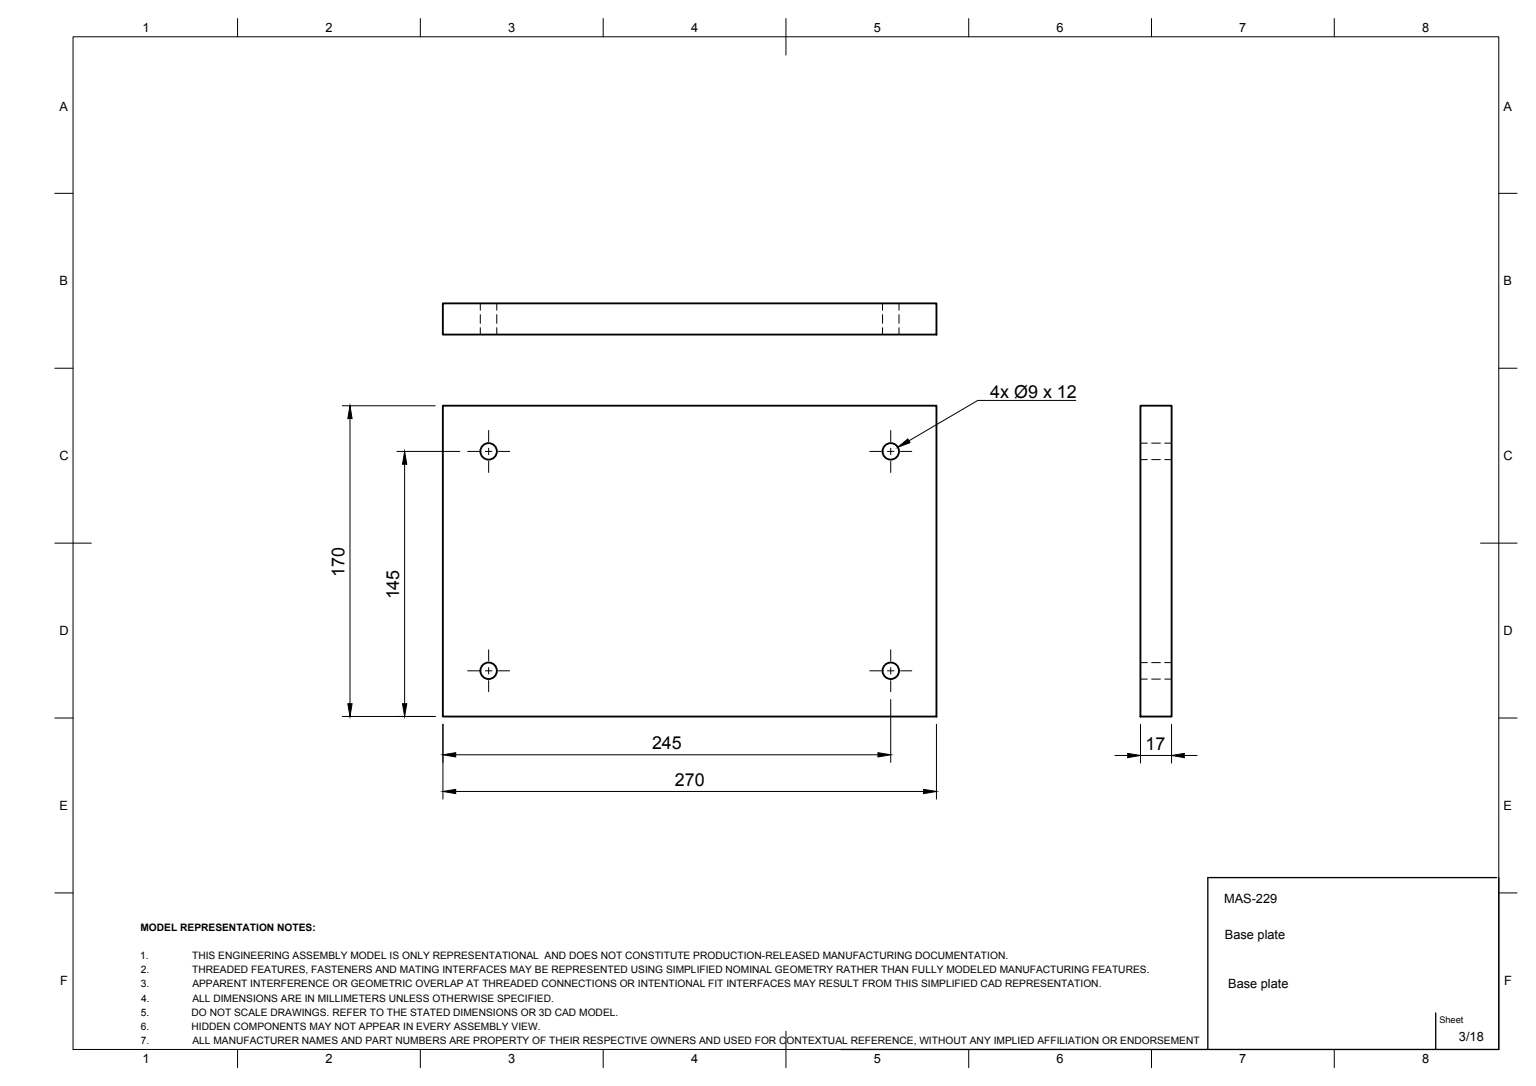
ISO-10303-21;
HEADER;
/* Generated by software containing ST-Developer
 * from STEP Tools, Inc. (www.steptools.com) 
 */

FILE_DESCRIPTION(
/* description */ ('Independently dimensioned six-bar single-leg walking-linkage demonstr
ator. Whole-mm20 crank,60 upper rocker,80/120 ternary coupler,120 lowe
r rocker,140 knee pitch and260 toe reach; ground pivots0/0,60/0,40/60.
 Seven native revolutes close both loops. Four reused native library f
amilies, fully retained shared pins and layered real spacer stacks, bo
nded rubber toe. Benchtop reference mechanism; no complete vehicle, lo
ad, gait stability, adhesive, weld, fit or life rating.'),
/* implementation_level */ '2;1');

FILE_NAME(
/* name */ 'Base plate.step',
/* time_stamp */ '2026-11-09T20:33:14-08:00',
/* author */ (''),
/* organization */ (''),
/* preprocessor_version */ 'ST-DEVELOPER v20.2',
/* originating_system */ 'Autodesk Translation Framework v15.17.0.0',
/* authorisation */ '');

FILE_SCHEMA (('AUTOMOTIVE_DESIGN { 1 0 10303 214 3 1 1 }'));
ENDSEC;

DATA;
#10=MECHANICAL_DESIGN_GEOMETRIC_PRESENTATION_REPRESENTATION('',(#255),#4048);
#219=SHAPE_REPRESENTATION_RELATIONSHIP('SRR','None',#4143,#237);
#237=ADVANCED_BREP_SHAPE_REPRESENTATION('',(#273),#4030);
#255=STYLED_ITEM('',(#4242),#273);
#273=MANIFOLD_SOLID_BREP('Body1',#2144);
#291=FACE_BOUND('',#550,.T.);
#292=FACE_BOUND('',#551,.T.);
#293=FACE_BOUND('',#552,.T.);
#294=FACE_BOUND('',#553,.T.);
#295=FACE_BOUND('',#555,.T.);
#296=FACE_BOUND('',#556,.T.);
#297=FACE_BOUND('',#557,.T.);
#298=FACE_BOUND('',#558,.T.);
#348=PLANE('',#2375);
#349=PLANE('',#2376);
#350=PLANE('',#2377);
#351=PLANE('',#2378);
#352=PLANE('',#2379);
#353=PLANE('',#2380);
#415=FACE_OUTER_BOUND('',#541,.T.);
#416=FACE_OUTER_BOUND('',#542,.T.);
#417=FACE_OUTER_BOUND('',#543,.T.);
#418=FACE_OUTER_BOUND('',#544,.T.);
#419=FACE_OUTER_BOUND('',#545,.T.);
#420=FACE_OUTER_BOUND('',#546,.T.);
#421=FACE_OUTER_BOUND('',#547,.T.);
#422=FACE_OUTER_BOUND('',#548,.T.);
#423=FACE_OUTER_BOUND('',#549,.T.);
#424=FACE_OUTER_BOUND('',#554,.T.);
#541=EDGE_LOOP('',(#1485,#1486,#1487,#1488));
#542=EDGE_LOOP('',(#1489,#1490,#1491,#1492));
#543=EDGE_LOOP('',(#1493,#1494,#1495,#1496));
#544=EDGE_LOOP('',(#1497,#1498,#1499,#1500));
#545=EDGE_LOOP('',(#1501,#1502,#1503,#1504));
#546=EDGE_LOOP('',(#1505,#1506,#1507,#1508));
#547=EDGE_LOOP('',(#1509,#1510,#1511,#1512));
#548=EDGE_LOOP('',(#1513,#1514,#1515,#1516));
#549=EDGE_LOOP('',(#1517,#1518,#1519,#1520));
#550=EDGE_LOOP('',(#1521));
#551=EDGE_LOOP('',(#1522));
#552=EDGE_LOOP('',(#1523));
#553=EDGE_LOOP('',(#1524));
#554=EDGE_LOOP('',(#1525,#1526,#1527,#1528));
#555=EDGE_LOOP('',(#1529));
#556=EDGE_LOOP('',(#1530));
#557=EDGE_LOOP('',(#1531));
#558=EDGE_LOOP('',(#1532));
#724=LINE('',#3422,#849);
#725=LINE('',#3428,#850);
#726=LINE('',#3434,#851);
#727=LINE('',#3440,#852);
#728=LINE('',#3445,#853);
#729=LINE('',#3447,#854);
#730=LINE('',#3449,#855);
#731=LINE('',#3450,#856);
#732=LINE('',#3453,#857);
#733=LINE('',#3455,#858);
#734=LINE('',#3456,#859);
#735=LINE('',#3459,#860);
#736=LINE('',#3461,#861);
#737=LINE('',#3462,#862);
#738=LINE('',#3464,#863);
#739=LINE('',#3465,#864);
#849=VECTOR('',#2679,4.5);
#850=VECTOR('',#2686,4.5);
#851=VECTOR('',#2693,4.5);
#852=VECTOR('',#2700,4.5);
#853=VECTOR('',#2705,10.);
#854=VECTOR('',#2706,10.);
#855=VECTOR('',#2707,10.);
#856=VECTOR('',#2708,10.);
#857=VECTOR('',#2711,10.);
#858=VECTOR('',#2712,10.);
#859=VECTOR('',#2713,10.);
#860=VECTOR('',#2716,10.);
#861=VECTOR('',#2717,10.);
#862=VECTOR('',#2718,10.);
#863=VECTOR('',#2721,10.);
#864=VECTOR('',#2722,10.);
#974=CIRCLE('',#2364,4.5);
#975=CIRCLE('',#2365,4.5);
#976=CIRCLE('',#2367,4.5);
#977=CIRCLE('',#2368,4.5);
#978=CIRCLE('',#2370,4.5);
#979=CIRCLE('',#2371,4.5);
#980=CIRCLE('',#2373,4.5);
#981=CIRCLE('',#2374,4.5);
#1088=VERTEX_POINT('',#3419);
#1089=VERTEX_POINT('',#3421);
#1090=VERTEX_POINT('',#3425);
#1091=VERTEX_POINT('',#3427);
#1092=VERTEX_POINT('',#3431);
#1093=VERTEX_POINT('',#3433);
#1094=VERTEX_POINT('',#3437);
#1095=VERTEX_POINT('',#3439);
#1096=VERTEX_POINT('',#3443);
#1097=VERTEX_POINT('',#3444);
#1098=VERTEX_POINT('',#3446);
#1099=VERTEX_POINT('',#3448);
#1100=VERTEX_POINT('',#3452);
#1101=VERTEX_POINT('',#3454);
#1102=VERTEX_POINT('',#3458);
#1103=VERTEX_POINT('',#3460);
#1246=EDGE_CURVE('',#1088,#1088,#974,.T.);
#1247=EDGE_CURVE('',#1088,#1089,#724,.T.);
#1248=EDGE_CURVE('',#1089,#1089,#975,.T.);
#1249=EDGE_CURVE('',#1090,#1090,#976,.T.);
#1250=EDGE_CURVE('',#1090,#1091,#725,.T.);
#1251=EDGE_CURVE('',#1091,#1091,#977,.T.);
#1252=EDGE_CURVE('',#1092,#1092,#978,.T.);
#1253=EDGE_CURVE('',#1092,#1093,#726,.T.);
#1254=EDGE_CURVE('',#1093,#1093,#979,.T.);
#1255=EDGE_CURVE('',#1094,#1094,#980,.T.);
#1256=EDGE_CURVE('',#1094,#1095,#727,.T.);
#1257=EDGE_CURVE('',#1095,#1095,#981,.T.);
#1258=EDGE_CURVE('',#1096,#1097,#728,.F.);
#1259=EDGE_CURVE('',#1097,#1098,#729,.T.);
#1260=EDGE_CURVE('',#1099,#1098,#730,.F.);
#1261=EDGE_CURVE('',#1096,#1099,#731,.T.);
#1262=EDGE_CURVE('',#1100,#1096,#732,.F.);
#1263=EDGE_CURVE('',#1101,#1099,#733,.F.);
#1264=EDGE_CURVE('',#1100,#1101,#734,.T.);
#1265=EDGE_CURVE('',#1102,#1100,#735,.F.);
#1266=EDGE_CURVE('',#1103,#1101,#736,.F.);
#1267=EDGE_CURVE('',#1102,#1103,#737,.F.);
#1268=EDGE_CURVE('',#1097,#1102,#738,.F.);
#1269=EDGE_CURVE('',#1098,#1103,#739,.F.);
#1485=ORIENTED_EDGE('',*,*,#1246,.F.);
#1486=ORIENTED_EDGE('',*,*,#1247,.T.);
#1487=ORIENTED_EDGE('',*,*,#1248,.F.);
#1488=ORIENTED_EDGE('',*,*,#1247,.F.);
#1489=ORIENTED_EDGE('',*,*,#1249,.F.);
#1490=ORIENTED_EDGE('',*,*,#1250,.T.);
#1491=ORIENTED_EDGE('',*,*,#1251,.F.);
#1492=ORIENTED_EDGE('',*,*,#1250,.F.);
#1493=ORIENTED_EDGE('',*,*,#1252,.F.);
#1494=ORIENTED_EDGE('',*,*,#1253,.T.);
#1495=ORIENTED_EDGE('',*,*,#1254,.F.);
#1496=ORIENTED_EDGE('',*,*,#1253,.F.);
#1497=ORIENTED_EDGE('',*,*,#1255,.F.);
#1498=ORIENTED_EDGE('',*,*,#1256,.T.);
#1499=ORIENTED_EDGE('',*,*,#1257,.F.);
#1500=ORIENTED_EDGE('',*,*,#1256,.F.);
#1501=ORIENTED_EDGE('',*,*,#1258,.T.);
#1502=ORIENTED_EDGE('',*,*,#1259,.T.);
#1503=ORIENTED_EDGE('',*,*,#1260,.F.);
#1504=ORIENTED_EDGE('',*,*,#1261,.F.);
#1505=ORIENTED_EDGE('',*,*,#1262,.T.);
#1506=ORIENTED_EDGE('',*,*,#1261,.T.);
#1507=ORIENTED_EDGE('',*,*,#1263,.F.);
#1508=ORIENTED_EDGE('',*,*,#1264,.F.);
#1509=ORIENTED_EDGE('',*,*,#1265,.T.);
#1510=ORIENTED_EDGE('',*,*,#1264,.T.);
#1511=ORIENTED_EDGE('',*,*,#1266,.F.);
#1512=ORIENTED_EDGE('',*,*,#1267,.F.);
#1513=ORIENTED_EDGE('',*,*,#1268,.T.);
#1514=ORIENTED_EDGE('',*,*,#1267,.T.);
#1515=ORIENTED_EDGE('',*,*,#1269,.F.);
#1516=ORIENTED_EDGE('',*,*,#1259,.F.);
#1517=ORIENTED_EDGE('',*,*,#1269,.T.);
#1518=ORIENTED_EDGE('',*,*,#1266,.T.);
#1519=ORIENTED_EDGE('',*,*,#1263,.T.);
#1520=ORIENTED_EDGE('',*,*,#1260,.T.);
#1521=ORIENTED_EDGE('',*,*,#1246,.T.);
#1522=ORIENTED_EDGE('',*,*,#1249,.T.);
#1523=ORIENTED_EDGE('',*,*,#1252,.T.);
#1524=ORIENTED_EDGE('',*,*,#1255,.T.);
#1525=ORIENTED_EDGE('',*,*,#1268,.F.);
#1526=ORIENTED_EDGE('',*,*,#1258,.F.);
#1527=ORIENTED_EDGE('',*,*,#1262,.F.);
#1528=ORIENTED_EDGE('',*,*,#1265,.F.);
#1529=ORIENTED_EDGE('',*,*,#1248,.T.);
#1530=ORIENTED_EDGE('',*,*,#1251,.T.);
#1531=ORIENTED_EDGE('',*,*,#1254,.T.);
#1532=ORIENTED_EDGE('',*,*,#1257,.T.);
#1963=CYLINDRICAL_SURFACE('',#2363,4.5);
#1964=CYLINDRICAL_SURFACE('',#2366,4.5);
#1965=CYLINDRICAL_SURFACE('',#2369,4.5);
#1966=CYLINDRICAL_SURFACE('',#2372,4.5);
#2018=ADVANCED_FACE('',(#415),#1963,.F.);
#2019=ADVANCED_FACE('',(#416),#1964,.F.);
#2020=ADVANCED_FACE('',(#417),#1965,.F.);
#2021=ADVANCED_FACE('',(#418),#1966,.F.);
#2022=ADVANCED_FACE('',(#419),#348,.T.);
#2023=ADVANCED_FACE('',(#420),#349,.T.);
#2024=ADVANCED_FACE('',(#421),#350,.T.);
#2025=ADVANCED_FACE('',(#422),#351,.T.);
#2026=ADVANCED_FACE('',(#423,#291,#292,#293,#294),#352,.T.);
#2027=ADVANCED_FACE('',(#424,#295,#296,#297,#298),#353,.F.);
#2144=CLOSED_SHELL('',(#2018,#2019,#2020,#2021,#2022,#2023,#2024,#2025,
#2026,#2027));
#2362=AXIS2_PLACEMENT_3D('',#3417,#2673,#2674);
#2363=AXIS2_PLACEMENT_3D('',#3418,#2675,#2676);
#2364=AXIS2_PLACEMENT_3D('',#3420,#2677,#2678);
#2365=AXIS2_PLACEMENT_3D('',#3423,#2680,#2681);
#2366=AXIS2_PLACEMENT_3D('',#3424,#2682,#2683);
#2367=AXIS2_PLACEMENT_3D('',#3426,#2684,#2685);
#2368=AXIS2_PLACEMENT_3D('',#3429,#2687,#2688);
#2369=AXIS2_PLACEMENT_3D('',#3430,#2689,#2690);
#2370=AXIS2_PLACEMENT_3D('',#3432,#2691,#2692);
#2371=AXIS2_PLACEMENT_3D('',#3435,#2694,#2695);
#2372=AXIS2_PLACEMENT_3D('',#3436,#2696,#2697);
#2373=AXIS2_PLACEMENT_3D('',#3438,#2698,#2699);
#2374=AXIS2_PLACEMENT_3D('',#3441,#2701,#2702);
#2375=AXIS2_PLACEMENT_3D('',#3442,#2703,#2704);
#2376=AXIS2_PLACEMENT_3D('',#3451,#2709,#2710);
#2377=AXIS2_PLACEMENT_3D('',#3457,#2714,#2715);
#2378=AXIS2_PLACEMENT_3D('',#3463,#2719,#2720);
#2379=AXIS2_PLACEMENT_3D('',#3466,#2723,#2724);
#2380=AXIS2_PLACEMENT_3D('',#3467,#2725,#2726);
#2673=DIRECTION('axis',(0.,0.,1.));
#2674=DIRECTION('refdir',(1.,0.,0.));
#2675=DIRECTION('center_axis',(0.,0.,-1.));
#2676=DIRECTION('ref_axis',(1.,0.,0.));
#2677=DIRECTION('center_axis',(0.,0.,-1.));
#2678=DIRECTION('ref_axis',(1.,0.,0.));
#2679=DIRECTION('',(0.,0.,-1.));
#2680=DIRECTION('center_axis',(0.,0.,1.));
#2681=DIRECTION('ref_axis',(1.,0.,0.));
#2682=DIRECTION('center_axis',(0.,0.,-1.));
#2683=DIRECTION('ref_axis',(1.,0.,0.));
#2684=DIRECTION('center_axis',(0.,0.,-1.));
#2685=DIRECTION('ref_axis',(1.,0.,0.));
#2686=DIRECTION('',(0.,0.,-1.));
#2687=DIRECTION('center_axis',(0.,0.,1.));
#2688=DIRECTION('ref_axis',(1.,0.,0.));
#2689=DIRECTION('center_axis',(0.,0.,-1.));
#2690=DIRECTION('ref_axis',(1.,0.,0.));
#2691=DIRECTION('center_axis',(0.,0.,-1.));
#2692=DIRECTION('ref_axis',(1.,0.,0.));
#2693=DIRECTION('',(0.,0.,-1.));
#2694=DIRECTION('center_axis',(0.,0.,1.));
#2695=DIRECTION('ref_axis',(1.,0.,0.));
#2696=DIRECTION('center_axis',(0.,0.,-1.));
#2697=DIRECTION('ref_axis',(1.,0.,0.));
#2698=DIRECTION('center_axis',(0.,0.,-1.));
#2699=DIRECTION('ref_axis',(1.,0.,0.));
#2700=DIRECTION('',(0.,0.,-1.));
#2701=DIRECTION('center_axis',(0.,0.,1.));
#2702=DIRECTION('ref_axis',(1.,0.,0.));
#2703=DIRECTION('center_axis',(0.,1.,0.));
#2704=DIRECTION('ref_axis',(-1.,0.,0.));
#2705=DIRECTION('',(1.,0.,0.));
#2706=DIRECTION('',(0.,0.,1.));
#2707=DIRECTION('',(1.,0.,0.));
#2708=DIRECTION('',(0.,0.,1.));
#2709=DIRECTION('center_axis',(1.,0.,0.));
#2710=DIRECTION('ref_axis',(0.,1.,0.));
#2711=DIRECTION('',(0.,-1.,0.));
#2712=DIRECTION('',(0.,-1.,0.));
#2713=DIRECTION('',(0.,0.,1.));
#2714=DIRECTION('center_axis',(0.,-1.,0.));
#2715=DIRECTION('ref_axis',(1.,0.,0.));
#2716=DIRECTION('',(-1.,0.,0.));
#2717=DIRECTION('',(-1.,0.,0.));
#2718=DIRECTION('',(0.,0.,-1.));
#2719=DIRECTION('center_axis',(-1.,0.,0.));
#2720=DIRECTION('ref_axis',(0.,-1.,0.));
#2721=DIRECTION('',(0.,1.,0.));
#2722=DIRECTION('',(0.,1.,0.));
#2723=DIRECTION('center_axis',(0.,0.,1.));
#2724=DIRECTION('ref_axis',(1.,0.,0.));
#2725=DIRECTION('center_axis',(0.,0.,1.));
#2726=DIRECTION('ref_axis',(1.,0.,0.));
#3417=CARTESIAN_POINT('',(0.,0.,0.));
#3418=CARTESIAN_POINT('Origin',(170.,-90.,6.));
#3419=CARTESIAN_POINT('',(165.5,-90.,12.));
#3420=CARTESIAN_POINT('Origin',(170.,-90.,12.));
#3421=CARTESIAN_POINT('',(165.5,-90.,-5.));
#3422=CARTESIAN_POINT('',(165.5,-90.,6.));
#3423=CARTESIAN_POINT('Origin',(170.,-90.,-5.));
#3424=CARTESIAN_POINT('Origin',(-50.,-90.,6.));
#3425=CARTESIAN_POINT('',(-54.5,-90.,12.));
#3426=CARTESIAN_POINT('Origin',(-50.,-90.,12.));
#3427=CARTESIAN_POINT('',(-54.5,-90.,-5.));
#3428=CARTESIAN_POINT('',(-54.5,-90.,6.));
#3429=CARTESIAN_POINT('Origin',(-50.,-90.,-5.));
#3430=CARTESIAN_POINT('Origin',(-50.,30.,6.));
#3431=CARTESIAN_POINT('',(-54.5,30.,12.));
#3432=CARTESIAN_POINT('Origin',(-50.,30.,12.));
#3433=CARTESIAN_POINT('',(-54.5,30.,-5.));
#3434=CARTESIAN_POINT('',(-54.5,30.,6.));
#3435=CARTESIAN_POINT('Origin',(-50.,30.,-5.));
#3436=CARTESIAN_POINT('Origin',(170.,30.,6.));
#3437=CARTESIAN_POINT('',(165.5,30.,12.));
#3438=CARTESIAN_POINT('Origin',(170.,30.,12.));
#3439=CARTESIAN_POINT('',(165.5,30.,-5.));
#3440=CARTESIAN_POINT('',(165.5,30.,6.));
#3441=CARTESIAN_POINT('Origin',(170.,30.,-5.));
#3442=CARTESIAN_POINT('Origin',(190.,55.,0.));
#3443=CARTESIAN_POINT('',(195.,55.,-5.));
#3444=CARTESIAN_POINT('',(-75.,55.,-5.));
#3445=CARTESIAN_POINT('',(125.,55.,-5.));
#3446=CARTESIAN_POINT('',(-75.,55.,12.));
#3447=CARTESIAN_POINT('',(-75.,55.,0.));
#3448=CARTESIAN_POINT('',(195.,55.,12.));
#3449=CARTESIAN_POINT('',(125.,55.,12.));
#3450=CARTESIAN_POINT('',(195.,55.,0.));
#3451=CARTESIAN_POINT('Origin',(195.,-110.,0.));
#3452=CARTESIAN_POINT('',(195.,-115.,-5.));
#3453=CARTESIAN_POINT('',(195.,-70.,-5.));
#3454=CARTESIAN_POINT('',(195.,-115.,12.));
#3455=CARTESIAN_POINT('',(195.,-70.,12.));
#3456=CARTESIAN_POINT('',(195.,-115.,0.));
#3457=CARTESIAN_POINT('Origin',(-70.,-115.,0.));
#3458=CARTESIAN_POINT('',(-75.,-115.,-5.));
#3459=CARTESIAN_POINT('',(-5.,-115.,-5.));
#3460=CARTESIAN_POINT('',(-75.,-115.,12.));
#3461=CARTESIAN_POINT('',(-5.,-115.,12.));
#3462=CARTESIAN_POINT('',(-75.,-115.,0.));
#3463=CARTESIAN_POINT('Origin',(-75.,50.,0.));
#3464=CARTESIAN_POINT('',(-75.,10.,-5.));
#3465=CARTESIAN_POINT('',(-75.,10.,12.));
#3466=CARTESIAN_POINT('Origin',(60.,-30.,12.));
#3467=CARTESIAN_POINT('Origin',(60.,-30.,-5.));
#4010=UNCERTAINTY_MEASURE_WITH_UNIT(LENGTH_MEASURE(0.01),#4049,
'DISTANCE_ACCURACY_VALUE',
'Maximum model space distance between geometric entities at asserted c
onnectivities');
#4028=UNCERTAINTY_MEASURE_WITH_UNIT(LENGTH_MEASURE(0.01),#4049,
'DISTANCE_ACCURACY_VALUE',
'Maximum model space distance between geometric entities at asserted c
onnectivities');
#4030=(
GEOMETRIC_REPRESENTATION_CONTEXT(3)
GLOBAL_UNCERTAINTY_ASSIGNED_CONTEXT((#4010))
GLOBAL_UNIT_ASSIGNED_CONTEXT((#4049,#4051,#4052))
REPRESENTATION_CONTEXT('','3D')
);
#4048=(
GEOMETRIC_REPRESENTATION_CONTEXT(3)
GLOBAL_UNCERTAINTY_ASSIGNED_CONTEXT((#4028))
GLOBAL_UNIT_ASSIGNED_CONTEXT((#4049,#4051,#4052))
REPRESENTATION_CONTEXT('','3D')
);
#4049=(
LENGTH_UNIT()
NAMED_UNIT(*)
SI_UNIT(.MILLI.,.METRE.)
);
#4051=(
NAMED_UNIT(*)
PLANE_ANGLE_UNIT()
SI_UNIT($,.RADIAN.)
);
#4052=(
NAMED_UNIT(*)
SI_UNIT($,.STERADIAN.)
SOLID_ANGLE_UNIT()
);
#4054=SHAPE_DEFINITION_REPRESENTATION(#4073,#4143);
#4073=PRODUCT_DEFINITION_SHAPE('',$,#4163);
#4143=SHAPE_REPRESENTATION('',(#2362),#4030);
#4161=PRODUCT_DEFINITION_CONTEXT('part definition',#4220,'design');
#4163=PRODUCT_DEFINITION('Base plate','Base plate',#4182,#4161);
#4182=PRODUCT_DEFINITION_FORMATION('',$,#4223);
#4220=APPLICATION_CONTEXT(
'Core Data for Automotive Mechanical Design Process');
#4221=PRODUCT_CONTEXT('part definition',#4220,'mechanical');
#4223=PRODUCT('Base plate','Base plate','Base plate',(#4221));
#4242=PRESENTATION_STYLE_ASSIGNMENT((#4256));
#4256=SURFACE_STYLE_USAGE(.BOTH.,#4270);
#4270=SURFACE_SIDE_STYLE('',(#4284));
#4284=SURFACE_STYLE_FILL_AREA(#4298);
#4298=FILL_AREA_STYLE('Dark blue',(#4312));
#4312=FILL_AREA_STYLE_COLOUR('Dark blue',#4326);
#4326=COLOUR_RGB('Dark blue',0.0901960784313725,0.270588235294118,0.513725490196078);
ENDSEC;
END-ISO-10303-21;
